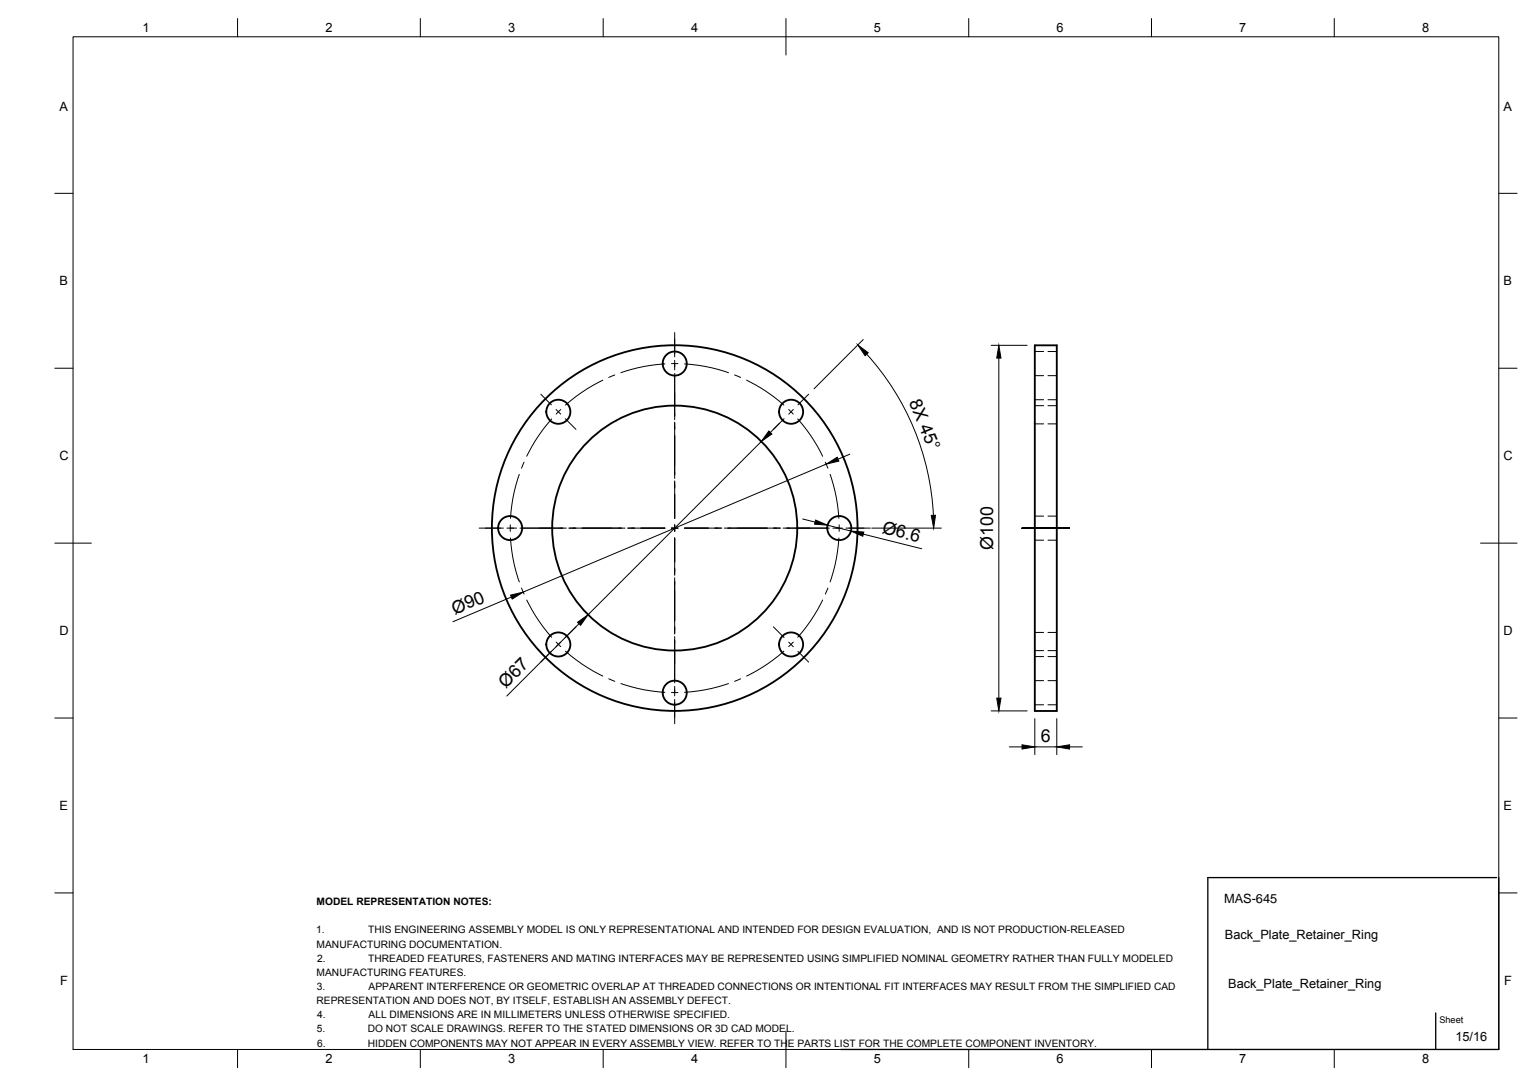
ISO-10303-21;
HEADER;
FILE_DESCRIPTION((''),'2;1');
FILE_NAME('Back_Plate_Retainer_Ring.step','2026-10-09T10:54:55-07:00',(''),(''),'','','');
FILE_SCHEMA (('AUTOMOTIVE_DESIGN { 1 0 10303 214 3 1 1 }'));
ENDSEC;
DATA;
#10=MECHANICAL_DESIGN_GEOMETRIC_PRESENTATION_REPRESENTATION('',(#608),#63824);
#578=SHAPE_REPRESENTATION_RELATIONSHIP('SRR','None',#63892,#593) ;
#593=ADVANCED_BREP_SHAPE_REPRESENTATION('',(#623),#63822) ;
#608=STYLED_ITEM('',(#63963),#623) ;
#623=MANIFOLD_SOLID_BREP('Body1',#15507) ;
#796=FACE_BOUND('',#3425,.T.) ;
#797=FACE_BOUND('',#3426,.T.) ;
#798=FACE_BOUND('',#3427,.T.) ;
#799=FACE_BOUND('',#3428,.T.) ;
#800=FACE_BOUND('',#3429,.T.) ;
#801=FACE_BOUND('',#3430,.T.) ;
#802=FACE_BOUND('',#3431,.T.) ;
#803=FACE_BOUND('',#3432,.T.) ;
#804=FACE_BOUND('',#3433,.T.) ;
#805=FACE_BOUND('',#3435,.T.) ;
#806=FACE_BOUND('',#3436,.T.) ;
#807=FACE_BOUND('',#3437,.T.) ;
#808=FACE_BOUND('',#3438,.T.) ;
#809=FACE_BOUND('',#3439,.T.) ;
#810=FACE_BOUND('',#3440,.T.) ;
#811=FACE_BOUND('',#3441,.T.) ;
#812=FACE_BOUND('',#3442,.T.) ;
#813=FACE_BOUND('',#3443,.T.) ;
#1112=PLANE('',#17850) ;
#1113=PLANE('',#17851) ;
#1525=CYLINDRICAL_SURFACE('',#17820,3.3) ;
#1526=CYLINDRICAL_SURFACE('',#17823,3.3) ;
#1527=CYLINDRICAL_SURFACE('',#17826,3.3) ;
#1528=CYLINDRICAL_SURFACE('',#17829,3.3) ;
#1529=CYLINDRICAL_SURFACE('',#17832,3.3) ;
#1530=CYLINDRICAL_SURFACE('',#17835,3.3) ;
#1531=CYLINDRICAL_SURFACE('',#17838,3.3) ;
#1532=CYLINDRICAL_SURFACE('',#17841,3.3) ;
#1533=CYLINDRICAL_SURFACE('',#17844,33.5) ;
#1534=CYLINDRICAL_SURFACE('',#17847,50.) ;
#2382=FACE_OUTER_BOUND('',#3414,.T.) ;
#2383=FACE_OUTER_BOUND('',#3415,.T.) ;
#2384=FACE_OUTER_BOUND('',#3416,.T.) ;
#2385=FACE_OUTER_BOUND('',#3417,.T.) ;
#2386=FACE_OUTER_BOUND('',#3418,.T.) ;
#2387=FACE_OUTER_BOUND('',#3419,.T.) ;
#2388=FACE_OUTER_BOUND('',#3420,.T.) ;
#2389=FACE_OUTER_BOUND('',#3421,.T.) ;
#2390=FACE_OUTER_BOUND('',#3422,.T.) ;
#2391=FACE_OUTER_BOUND('',#3423,.T.) ;
#2392=FACE_OUTER_BOUND('',#3424,.T.) ;
#2393=FACE_OUTER_BOUND('',#3434,.T.) ;
#3414=EDGE_LOOP('',(#14376,#14377,#14378,#14379)) ;
#3415=EDGE_LOOP('',(#14380,#14381,#14382,#14383)) ;
#3416=EDGE_LOOP('',(#14384,#14385,#14386,#14387)) ;
#3417=EDGE_LOOP('',(#14388,#14389,#14390,#14391)) ;
#3418=EDGE_LOOP('',(#14392,#14393,#14394,#14395)) ;
#3419=EDGE_LOOP('',(#14396,#14397,#14398,#14399)) ;
#3420=EDGE_LOOP('',(#14400,#14401,#14402,#14403)) ;
#3421=EDGE_LOOP('',(#14404,#14405,#14406,#14407)) ;
#3422=EDGE_LOOP('',(#14408,#14409,#14410,#14411)) ;
#3423=EDGE_LOOP('',(#14412,#14413,#14414,#14415)) ;
#3424=EDGE_LOOP('',(#14416)) ;
#3425=EDGE_LOOP('',(#14417)) ;
#3426=EDGE_LOOP('',(#14418)) ;
#3427=EDGE_LOOP('',(#14419)) ;
#3428=EDGE_LOOP('',(#14420)) ;
#3429=EDGE_LOOP('',(#14421)) ;
#3430=EDGE_LOOP('',(#14422)) ;
#3431=EDGE_LOOP('',(#14423)) ;
#3432=EDGE_LOOP('',(#14424)) ;
#3433=EDGE_LOOP('',(#14425)) ;
#3434=EDGE_LOOP('',(#14426)) ;
#3435=EDGE_LOOP('',(#14427)) ;
#3436=EDGE_LOOP('',(#14428)) ;
#3437=EDGE_LOOP('',(#14429)) ;
#3438=EDGE_LOOP('',(#14430)) ;
#3439=EDGE_LOOP('',(#14431)) ;
#3440=EDGE_LOOP('',(#14432)) ;
#3441=EDGE_LOOP('',(#14433)) ;
#3442=EDGE_LOOP('',(#14434)) ;
#3443=EDGE_LOOP('',(#14435)) ;
#4650=CIRCLE('',#17821,3.3) ;
#4651=CIRCLE('',#17822,3.3) ;
#4652=CIRCLE('',#17824,3.3) ;
#4653=CIRCLE('',#17825,3.3) ;
#4654=CIRCLE('',#17827,3.3) ;
#4655=CIRCLE('',#17828,3.3) ;
#4656=CIRCLE('',#17830,3.3) ;
#4657=CIRCLE('',#17831,3.3) ;
#4658=CIRCLE('',#17833,3.3) ;
#4659=CIRCLE('',#17834,3.3) ;
#4660=CIRCLE('',#17836,3.3) ;
#4661=CIRCLE('',#17837,3.3) ;
#4662=CIRCLE('',#17839,3.3) ;
#4663=CIRCLE('',#17840,3.3) ;
#4664=CIRCLE('',#17842,3.3) ;
#4665=CIRCLE('',#17843,3.3) ;
#4666=CIRCLE('',#17845,33.5) ;
#4667=CIRCLE('',#17846,33.5) ;
#4668=CIRCLE('',#17848,50.) ;
#4669=CIRCLE('',#17849,50.) ;
#5326=LINE('',#63653,#5982) ;
#5327=LINE('',#63659,#5983) ;
#5328=LINE('',#63665,#5984) ;
#5329=LINE('',#63671,#5985) ;
#5330=LINE('',#63677,#5986) ;
#5331=LINE('',#63683,#5987) ;
#5332=LINE('',#63689,#5988) ;
#5333=LINE('',#63695,#5989) ;
#5334=LINE('',#63701,#5990) ;
#5335=LINE('',#63707,#5991) ;
#5982=VECTOR('',#22832,3.3) ;
#5983=VECTOR('',#22839,3.3) ;
#5984=VECTOR('',#22846,3.3) ;
#5985=VECTOR('',#22853,3.3) ;
#5986=VECTOR('',#22860,3.3) ;
#5987=VECTOR('',#22867,3.3) ;
#5988=VECTOR('',#22874,3.3) ;
#5989=VECTOR('',#22881,3.3) ;
#5990=VECTOR('',#22888,33.5) ;
#5991=VECTOR('',#22895,50.) ;
#7415=VERTEX_POINT('',#63650) ;
#7416=VERTEX_POINT('',#63652) ;
#7417=VERTEX_POINT('',#63656) ;
#7418=VERTEX_POINT('',#63658) ;
#7419=VERTEX_POINT('',#63662) ;
#7420=VERTEX_POINT('',#63664) ;
#7421=VERTEX_POINT('',#63668) ;
#7422=VERTEX_POINT('',#63670) ;
#7423=VERTEX_POINT('',#63674) ;
#7424=VERTEX_POINT('',#63676) ;
#7425=VERTEX_POINT('',#63680) ;
#7426=VERTEX_POINT('',#63682) ;
#7427=VERTEX_POINT('',#63686) ;
#7428=VERTEX_POINT('',#63688) ;
#7429=VERTEX_POINT('',#63692) ;
#7430=VERTEX_POINT('',#63694) ;
#7431=VERTEX_POINT('',#63698) ;
#7432=VERTEX_POINT('',#63700) ;
#7433=VERTEX_POINT('',#63704) ;
#7434=VERTEX_POINT('',#63706) ;
#9742=EDGE_CURVE('',#7415,#7415,#4650,.T.) ;
#9743=EDGE_CURVE('',#7415,#7416,#5326,.T.) ;
#9744=EDGE_CURVE('',#7416,#7416,#4651,.T.) ;
#9745=EDGE_CURVE('',#7417,#7417,#4652,.T.) ;
#9746=EDGE_CURVE('',#7417,#7418,#5327,.T.) ;
#9747=EDGE_CURVE('',#7418,#7418,#4653,.T.) ;
#9748=EDGE_CURVE('',#7419,#7419,#4654,.T.) ;
#9749=EDGE_CURVE('',#7419,#7420,#5328,.T.) ;
#9750=EDGE_CURVE('',#7420,#7420,#4655,.T.) ;
#9751=EDGE_CURVE('',#7421,#7421,#4656,.T.) ;
#9752=EDGE_CURVE('',#7421,#7422,#5329,.T.) ;
#9753=EDGE_CURVE('',#7422,#7422,#4657,.T.) ;
#9754=EDGE_CURVE('',#7423,#7423,#4658,.T.) ;
#9755=EDGE_CURVE('',#7423,#7424,#5330,.T.) ;
#9756=EDGE_CURVE('',#7424,#7424,#4659,.T.) ;
#9757=EDGE_CURVE('',#7425,#7425,#4660,.T.) ;
#9758=EDGE_CURVE('',#7425,#7426,#5331,.T.) ;
#9759=EDGE_CURVE('',#7426,#7426,#4661,.T.) ;
#9760=EDGE_CURVE('',#7427,#7427,#4662,.T.) ;
#9761=EDGE_CURVE('',#7427,#7428,#5332,.T.) ;
#9762=EDGE_CURVE('',#7428,#7428,#4663,.T.) ;
#9763=EDGE_CURVE('',#7429,#7429,#4664,.T.) ;
#9764=EDGE_CURVE('',#7429,#7430,#5333,.T.) ;
#9765=EDGE_CURVE('',#7430,#7430,#4665,.T.) ;
#9766=EDGE_CURVE('',#7431,#7431,#4666,.T.) ;
#9767=EDGE_CURVE('',#7431,#7432,#5334,.T.) ;
#9768=EDGE_CURVE('',#7432,#7432,#4667,.T.) ;
#9769=EDGE_CURVE('',#7433,#7433,#4668,.T.) ;
#9770=EDGE_CURVE('',#7433,#7434,#5335,.T.) ;
#9771=EDGE_CURVE('',#7434,#7434,#4669,.T.) ;
#14376=ORIENTED_EDGE('',*,*,#9742,.F.) ;
#14377=ORIENTED_EDGE('',*,*,#9743,.T.) ;
#14378=ORIENTED_EDGE('',*,*,#9744,.F.) ;
#14379=ORIENTED_EDGE('',*,*,#9743,.F.) ;
#14380=ORIENTED_EDGE('',*,*,#9745,.F.) ;
#14381=ORIENTED_EDGE('',*,*,#9746,.T.) ;
#14382=ORIENTED_EDGE('',*,*,#9747,.F.) ;
#14383=ORIENTED_EDGE('',*,*,#9746,.F.) ;
#14384=ORIENTED_EDGE('',*,*,#9748,.F.) ;
#14385=ORIENTED_EDGE('',*,*,#9749,.T.) ;
#14386=ORIENTED_EDGE('',*,*,#9750,.F.) ;
#14387=ORIENTED_EDGE('',*,*,#9749,.F.) ;
#14388=ORIENTED_EDGE('',*,*,#9751,.F.) ;
#14389=ORIENTED_EDGE('',*,*,#9752,.T.) ;
#14390=ORIENTED_EDGE('',*,*,#9753,.F.) ;
#14391=ORIENTED_EDGE('',*,*,#9752,.F.) ;
#14392=ORIENTED_EDGE('',*,*,#9754,.F.) ;
#14393=ORIENTED_EDGE('',*,*,#9755,.T.) ;
#14394=ORIENTED_EDGE('',*,*,#9756,.F.) ;
#14395=ORIENTED_EDGE('',*,*,#9755,.F.) ;
#14396=ORIENTED_EDGE('',*,*,#9757,.F.) ;
#14397=ORIENTED_EDGE('',*,*,#9758,.T.) ;
#14398=ORIENTED_EDGE('',*,*,#9759,.F.) ;
#14399=ORIENTED_EDGE('',*,*,#9758,.F.) ;
#14400=ORIENTED_EDGE('',*,*,#9760,.F.) ;
#14401=ORIENTED_EDGE('',*,*,#9761,.T.) ;
#14402=ORIENTED_EDGE('',*,*,#9762,.F.) ;
#14403=ORIENTED_EDGE('',*,*,#9761,.F.) ;
#14404=ORIENTED_EDGE('',*,*,#9763,.F.) ;
#14405=ORIENTED_EDGE('',*,*,#9764,.T.) ;
#14406=ORIENTED_EDGE('',*,*,#9765,.F.) ;
#14407=ORIENTED_EDGE('',*,*,#9764,.F.) ;
#14408=ORIENTED_EDGE('',*,*,#9766,.F.) ;
#14409=ORIENTED_EDGE('',*,*,#9767,.T.) ;
#14410=ORIENTED_EDGE('',*,*,#9768,.F.) ;
#14411=ORIENTED_EDGE('',*,*,#9767,.F.) ;
#14412=ORIENTED_EDGE('',*,*,#9769,.F.) ;
#14413=ORIENTED_EDGE('',*,*,#9770,.T.) ;
#14414=ORIENTED_EDGE('',*,*,#9771,.F.) ;
#14415=ORIENTED_EDGE('',*,*,#9770,.F.) ;
#14416=ORIENTED_EDGE('',*,*,#9771,.T.) ;
#14417=ORIENTED_EDGE('',*,*,#9744,.T.) ;
#14418=ORIENTED_EDGE('',*,*,#9747,.T.) ;
#14419=ORIENTED_EDGE('',*,*,#9750,.T.) ;
#14420=ORIENTED_EDGE('',*,*,#9753,.T.) ;
#14421=ORIENTED_EDGE('',*,*,#9756,.T.) ;
#14422=ORIENTED_EDGE('',*,*,#9759,.T.) ;
#14423=ORIENTED_EDGE('',*,*,#9762,.T.) ;
#14424=ORIENTED_EDGE('',*,*,#9765,.T.) ;
#14425=ORIENTED_EDGE('',*,*,#9766,.T.) ;
#14426=ORIENTED_EDGE('',*,*,#9769,.T.) ;
#14427=ORIENTED_EDGE('',*,*,#9742,.T.) ;
#14428=ORIENTED_EDGE('',*,*,#9745,.T.) ;
#14429=ORIENTED_EDGE('',*,*,#9748,.T.) ;
#14430=ORIENTED_EDGE('',*,*,#9751,.T.) ;
#14431=ORIENTED_EDGE('',*,*,#9754,.T.) ;
#14432=ORIENTED_EDGE('',*,*,#9757,.T.) ;
#14433=ORIENTED_EDGE('',*,*,#9760,.T.) ;
#14434=ORIENTED_EDGE('',*,*,#9763,.T.) ;
#14435=ORIENTED_EDGE('',*,*,#9768,.T.) ;
#15470=ADVANCED_FACE('',(#2382),#1525,.F.) ;
#15471=ADVANCED_FACE('',(#2383),#1526,.F.) ;
#15472=ADVANCED_FACE('',(#2384),#1527,.F.) ;
#15473=ADVANCED_FACE('',(#2385),#1528,.F.) ;
#15474=ADVANCED_FACE('',(#2386),#1529,.F.) ;
#15475=ADVANCED_FACE('',(#2387),#1530,.F.) ;
#15476=ADVANCED_FACE('',(#2388),#1531,.F.) ;
#15477=ADVANCED_FACE('',(#2389),#1532,.F.) ;
#15478=ADVANCED_FACE('',(#2390),#1533,.F.) ;
#15479=ADVANCED_FACE('',(#2391),#1534,.T.) ;
#15480=ADVANCED_FACE('',(#2392,#796,#797,#798,#799,#800,#801,#802,#803,
#804),#1112,.F.) ;
#15481=ADVANCED_FACE('',(#2393,#805,#806,#807,#808,#809,#810,#811,#812,
#813),#1113,.T.) ;
#15507=CLOSED_SHELL('',(#15470,#15471,#15472,#15473,#15474,#15475,#15476,
#15477,#15478,#15479,#15480,#15481)) ;
#17819=AXIS2_PLACEMENT_3D('',#63648,#22826,#22827) ;
#17820=AXIS2_PLACEMENT_3D('',#63649,#22828,#22829) ;
#17821=AXIS2_PLACEMENT_3D('',#63651,#22830,#22831) ;
#17822=AXIS2_PLACEMENT_3D('',#63654,#22833,#22834) ;
#17823=AXIS2_PLACEMENT_3D('',#63655,#22835,#22836) ;
#17824=AXIS2_PLACEMENT_3D('',#63657,#22837,#22838) ;
#17825=AXIS2_PLACEMENT_3D('',#63660,#22840,#22841) ;
#17826=AXIS2_PLACEMENT_3D('',#63661,#22842,#22843) ;
#17827=AXIS2_PLACEMENT_3D('',#63663,#22844,#22845) ;
#17828=AXIS2_PLACEMENT_3D('',#63666,#22847,#22848) ;
#17829=AXIS2_PLACEMENT_3D('',#63667,#22849,#22850) ;
#17830=AXIS2_PLACEMENT_3D('',#63669,#22851,#22852) ;
#17831=AXIS2_PLACEMENT_3D('',#63672,#22854,#22855) ;
#17832=AXIS2_PLACEMENT_3D('',#63673,#22856,#22857) ;
#17833=AXIS2_PLACEMENT_3D('',#63675,#22858,#22859) ;
#17834=AXIS2_PLACEMENT_3D('',#63678,#22861,#22862) ;
#17835=AXIS2_PLACEMENT_3D('',#63679,#22863,#22864) ;
#17836=AXIS2_PLACEMENT_3D('',#63681,#22865,#22866) ;
#17837=AXIS2_PLACEMENT_3D('',#63684,#22868,#22869) ;
#17838=AXIS2_PLACEMENT_3D('',#63685,#22870,#22871) ;
#17839=AXIS2_PLACEMENT_3D('',#63687,#22872,#22873) ;
#17840=AXIS2_PLACEMENT_3D('',#63690,#22875,#22876) ;
#17841=AXIS2_PLACEMENT_3D('',#63691,#22877,#22878) ;
#17842=AXIS2_PLACEMENT_3D('',#63693,#22879,#22880) ;
#17843=AXIS2_PLACEMENT_3D('',#63696,#22882,#22883) ;
#17844=AXIS2_PLACEMENT_3D('',#63697,#22884,#22885) ;
#17845=AXIS2_PLACEMENT_3D('',#63699,#22886,#22887) ;
#17846=AXIS2_PLACEMENT_3D('',#63702,#22889,#22890) ;
#17847=AXIS2_PLACEMENT_3D('',#63703,#22891,#22892) ;
#17848=AXIS2_PLACEMENT_3D('',#63705,#22893,#22894) ;
#17849=AXIS2_PLACEMENT_3D('',#63708,#22896,#22897) ;
#17850=AXIS2_PLACEMENT_3D('',#63709,#22898,#22899) ;
#17851=AXIS2_PLACEMENT_3D('',#63710,#22900,#22901) ;
#22826=DIRECTION('axis',(0.,0.,1.)) ;
#22827=DIRECTION('refdir',(1.,0.,0.)) ;
#22828=DIRECTION('center_axis',(0.,0.,1.)) ;
#22829=DIRECTION('ref_axis',(-1.,0.,0.)) ;
#22830=DIRECTION('center_axis',(0.,0.,1.)) ;
#22831=DIRECTION('ref_axis',(-1.,0.,0.)) ;
#22832=DIRECTION('',(0.,0.,1.)) ;
#22833=DIRECTION('center_axis',(0.,0.,-1.)) ;
#22834=DIRECTION('ref_axis',(-1.,0.,0.)) ;
#22835=DIRECTION('center_axis',(0.,0.,1.)) ;
#22836=DIRECTION('ref_axis',(-1.,0.,0.)) ;
#22837=DIRECTION('center_axis',(0.,0.,1.)) ;
#22838=DIRECTION('ref_axis',(-1.,0.,0.)) ;
#22839=DIRECTION('',(0.,0.,1.)) ;
#22840=DIRECTION('center_axis',(0.,0.,-1.)) ;
#22841=DIRECTION('ref_axis',(-1.,0.,0.)) ;
#22842=DIRECTION('center_axis',(0.,0.,1.)) ;
#22843=DIRECTION('ref_axis',(-1.,0.,0.)) ;
#22844=DIRECTION('center_axis',(0.,0.,1.)) ;
#22845=DIRECTION('ref_axis',(-1.,0.,0.)) ;
#22846=DIRECTION('',(0.,0.,1.)) ;
#22847=DIRECTION('center_axis',(0.,0.,-1.)) ;
#22848=DIRECTION('ref_axis',(-1.,0.,0.)) ;
#22849=DIRECTION('center_axis',(0.,0.,1.)) ;
#22850=DIRECTION('ref_axis',(-1.,0.,0.)) ;
#22851=DIRECTION('center_axis',(0.,0.,1.)) ;
#22852=DIRECTION('ref_axis',(-1.,0.,0.)) ;
#22853=DIRECTION('',(0.,0.,1.)) ;
#22854=DIRECTION('center_axis',(0.,0.,-1.)) ;
#22855=DIRECTION('ref_axis',(-1.,0.,0.)) ;
#22856=DIRECTION('center_axis',(0.,0.,1.)) ;
#22857=DIRECTION('ref_axis',(-1.,0.,0.)) ;
#22858=DIRECTION('center_axis',(0.,0.,1.)) ;
#22859=DIRECTION('ref_axis',(-1.,0.,0.)) ;
#22860=DIRECTION('',(0.,0.,1.)) ;
#22861=DIRECTION('center_axis',(0.,0.,-1.)) ;
#22862=DIRECTION('ref_axis',(-1.,0.,0.)) ;
#22863=DIRECTION('center_axis',(0.,0.,1.)) ;
#22864=DIRECTION('ref_axis',(-1.,0.,0.)) ;
#22865=DIRECTION('center_axis',(0.,0.,1.)) ;
#22866=DIRECTION('ref_axis',(-1.,0.,0.)) ;
#22867=DIRECTION('',(0.,0.,1.)) ;
#22868=DIRECTION('center_axis',(0.,0.,-1.)) ;
#22869=DIRECTION('ref_axis',(-1.,0.,0.)) ;
#22870=DIRECTION('center_axis',(0.,0.,1.)) ;
#22871=DIRECTION('ref_axis',(-1.,0.,0.)) ;
#22872=DIRECTION('center_axis',(0.,0.,1.)) ;
#22873=DIRECTION('ref_axis',(-1.,0.,0.)) ;
#22874=DIRECTION('',(0.,0.,1.)) ;
#22875=DIRECTION('center_axis',(0.,0.,-1.)) ;
#22876=DIRECTION('ref_axis',(-1.,0.,0.)) ;
#22877=DIRECTION('center_axis',(0.,0.,1.)) ;
#22878=DIRECTION('ref_axis',(-1.,0.,0.)) ;
#22879=DIRECTION('center_axis',(0.,0.,1.)) ;
#22880=DIRECTION('ref_axis',(-1.,0.,0.)) ;
#22881=DIRECTION('',(0.,0.,1.)) ;
#22882=DIRECTION('center_axis',(0.,0.,-1.)) ;
#22883=DIRECTION('ref_axis',(-1.,0.,0.)) ;
#22884=DIRECTION('center_axis',(0.,0.,-1.)) ;
#22885=DIRECTION('ref_axis',(1.,0.,0.)) ;
#22886=DIRECTION('center_axis',(0.,0.,-1.)) ;
#22887=DIRECTION('ref_axis',(1.,0.,0.)) ;
#22888=DIRECTION('',(0.,0.,-1.)) ;
#22889=DIRECTION('center_axis',(0.,0.,1.)) ;
#22890=DIRECTION('ref_axis',(1.,0.,0.)) ;
#22891=DIRECTION('center_axis',(0.,0.,-1.)) ;
#22892=DIRECTION('ref_axis',(1.,0.,0.)) ;
#22893=DIRECTION('center_axis',(0.,0.,-1.)) ;
#22894=DIRECTION('ref_axis',(1.,0.,0.)) ;
#22895=DIRECTION('',(0.,0.,1.)) ;
#22896=DIRECTION('center_axis',(0.,0.,1.)) ;
#22897=DIRECTION('ref_axis',(1.,0.,0.)) ;
#22898=DIRECTION('center_axis',(0.,0.,-1.)) ;
#22899=DIRECTION('ref_axis',(-1.,0.,0.)) ;
#22900=DIRECTION('center_axis',(0.,0.,-1.)) ;
#22901=DIRECTION('ref_axis',(-1.,0.,0.)) ;
#63648=CARTESIAN_POINT('',(0.,0.,0.)) ;
#63649=CARTESIAN_POINT('Origin',(45.,354.45,-22.)) ;
#63650=CARTESIAN_POINT('',(48.3,354.45,-30.)) ;
#63651=CARTESIAN_POINT('Origin',(45.,354.45,-30.)) ;
#63652=CARTESIAN_POINT('',(48.3,354.45,-24.)) ;
#63653=CARTESIAN_POINT('',(48.3,354.45,-22.)) ;
#63654=CARTESIAN_POINT('Origin',(45.,354.45,-24.)) ;
#63655=CARTESIAN_POINT('Origin',(-5.51091059616309E-15,399.45,-22.)) ;
#63656=CARTESIAN_POINT('',(3.29999999999999,399.45,-30.)) ;
#63657=CARTESIAN_POINT('Origin',(-5.51091059616309E-15,399.45,-30.)) ;
#63658=CARTESIAN_POINT('',(3.29999999999999,399.45,-24.)) ;
#63659=CARTESIAN_POINT('',(3.29999999999999,399.45,-22.)) ;
#63660=CARTESIAN_POINT('Origin',(-5.51091059616309E-15,399.45,-24.)) ;
#63661=CARTESIAN_POINT('Origin',(-45.,354.45,-22.)) ;
#63662=CARTESIAN_POINT('',(-41.7,354.45,-30.)) ;
#63663=CARTESIAN_POINT('Origin',(-45.,354.45,-30.)) ;
#63664=CARTESIAN_POINT('',(-41.7,354.45,-24.)) ;
#63665=CARTESIAN_POINT('',(-41.7,354.45,-22.)) ;
#63666=CARTESIAN_POINT('Origin',(-45.,354.45,-24.)) ;
#63667=CARTESIAN_POINT('Origin',(0.,309.45,-22.)) ;
#63668=CARTESIAN_POINT('',(3.3,309.45,-30.)) ;
#63669=CARTESIAN_POINT('Origin',(0.,309.45,-30.)) ;
#63670=CARTESIAN_POINT('',(3.3,309.45,-24.)) ;
#63671=CARTESIAN_POINT('',(3.3,309.45,-22.)) ;
#63672=CARTESIAN_POINT('Origin',(0.,309.45,-24.)) ;
#63673=CARTESIAN_POINT('Origin',(-31.8198051533946,322.630194846605,-22.)) ;
#63674=CARTESIAN_POINT('',(-28.5198051533946,322.630194846605,-30.)) ;
#63675=CARTESIAN_POINT('Origin',(-31.8198051533946,322.630194846605,-30.)) ;
#63676=CARTESIAN_POINT('',(-28.5198051533946,322.630194846605,-24.)) ;
#63677=CARTESIAN_POINT('',(-28.5198051533946,322.630194846605,-22.)) ;
#63678=CARTESIAN_POINT('Origin',(-31.8198051533946,322.630194846605,-24.)) ;
#63679=CARTESIAN_POINT('Origin',(-31.8198051533946,386.269805153395,-22.)) ;
#63680=CARTESIAN_POINT('',(-28.5198051533946,386.269805153395,-30.)) ;
#63681=CARTESIAN_POINT('Origin',(-31.8198051533946,386.269805153395,-30.)) ;
#63682=CARTESIAN_POINT('',(-28.5198051533946,386.269805153395,-24.)) ;
#63683=CARTESIAN_POINT('',(-28.5198051533946,386.269805153395,-22.)) ;
#63684=CARTESIAN_POINT('Origin',(-31.8198051533946,386.269805153395,-24.)) ;
#63685=CARTESIAN_POINT('Origin',(31.8198051533946,386.269805153395,-22.)) ;
#63686=CARTESIAN_POINT('',(35.1198051533946,386.269805153395,-30.)) ;
#63687=CARTESIAN_POINT('Origin',(31.8198051533946,386.269805153395,-30.)) ;
#63688=CARTESIAN_POINT('',(35.1198051533946,386.269805153395,-24.)) ;
#63689=CARTESIAN_POINT('',(35.1198051533946,386.269805153395,-22.)) ;
#63690=CARTESIAN_POINT('Origin',(31.8198051533946,386.269805153395,-24.)) ;
#63691=CARTESIAN_POINT('Origin',(31.8198051533946,322.630194846605,-22.)) ;
#63692=CARTESIAN_POINT('',(35.1198051533946,322.630194846605,-30.)) ;
#63693=CARTESIAN_POINT('Origin',(31.8198051533946,322.630194846605,-30.)) ;
#63694=CARTESIAN_POINT('',(35.1198051533946,322.630194846605,-24.)) ;
#63695=CARTESIAN_POINT('',(35.1198051533946,322.630194846605,-22.)) ;
#63696=CARTESIAN_POINT('Origin',(31.8198051533946,322.630194846605,-24.)) ;
#63697=CARTESIAN_POINT('Origin',(0.,354.45,-24.)) ;
#63698=CARTESIAN_POINT('',(-33.5,354.45,-24.)) ;
#63699=CARTESIAN_POINT('Origin',(0.,354.45,-24.)) ;
#63700=CARTESIAN_POINT('',(-33.5,354.45,-30.)) ;
#63701=CARTESIAN_POINT('',(-33.5,354.45,-24.)) ;
#63702=CARTESIAN_POINT('Origin',(0.,354.45,-30.)) ;
#63703=CARTESIAN_POINT('Origin',(0.,354.45,-24.)) ;
#63704=CARTESIAN_POINT('',(-50.,354.45,-30.)) ;
#63705=CARTESIAN_POINT('Origin',(0.,354.45,-30.)) ;
#63706=CARTESIAN_POINT('',(-50.,354.45,-24.)) ;
#63707=CARTESIAN_POINT('',(-50.,354.45,-24.)) ;
#63708=CARTESIAN_POINT('Origin',(0.,354.45,-24.)) ;
#63709=CARTESIAN_POINT('Origin',(0.,354.45,-24.)) ;
#63710=CARTESIAN_POINT('Origin',(0.,354.45,-30.)) ;
#63805=UNCERTAINTY_MEASURE_WITH_UNIT(LENGTH_MEASURE(0.01),#63825,
'DISTANCE_ACCURACY_VALUE',
'Maximum model space distance between geometric entities at asserted c
onnectivities') ;
#63807=UNCERTAINTY_MEASURE_WITH_UNIT(LENGTH_MEASURE(0.01),#63825,
'DISTANCE_ACCURACY_VALUE',
'Maximum model space distance between geometric entities at asserted c
onnectivities') ;
#63822=(
GEOMETRIC_REPRESENTATION_CONTEXT(3)
GLOBAL_UNCERTAINTY_ASSIGNED_CONTEXT((#63805))
GLOBAL_UNIT_ASSIGNED_CONTEXT((#63825,#63827,#63828))
REPRESENTATION_CONTEXT('','3D')
) ;
#63824=(
GEOMETRIC_REPRESENTATION_CONTEXT(3)
GLOBAL_UNCERTAINTY_ASSIGNED_CONTEXT((#63807))
GLOBAL_UNIT_ASSIGNED_CONTEXT((#63825,#63827,#63828))
REPRESENTATION_CONTEXT('','3D')
) ;
#63825=(
LENGTH_UNIT()
NAMED_UNIT(*)
SI_UNIT(.MILLI.,.METRE.)
) ;
#63827=(
NAMED_UNIT(*)
PLANE_ANGLE_UNIT()
SI_UNIT($,.RADIAN.)
) ;
#63828=(
NAMED_UNIT(*)
SI_UNIT($,.STERADIAN.)
SOLID_ANGLE_UNIT()
) ;
#63843=SHAPE_DEFINITION_REPRESENTATION(#63859,#63892) ;
#63859=PRODUCT_DEFINITION_SHAPE('',$,#63909) ;
#63892=SHAPE_REPRESENTATION('',(#17819),#63822) ;
#63894=PRODUCT_DEFINITION_CONTEXT('part definition',#63944,'design') ;
#63909=PRODUCT_DEFINITION('Back_Plate_Retainer_Ring',
'Back_Plate_Retainer_Ring',#63925,#63894) ;
#63925=PRODUCT_DEFINITION_FORMATION('',$,#63960) ;
#63944=APPLICATION_CONTEXT(
'Core Data for Automotive Mechanical Design Process') ;
#63945=PRODUCT_CONTEXT('part definition',#63944,'mechanical') ;
#63960=PRODUCT('Back_Plate_Retainer_Ring','Back_Plate_Retainer_Ring',$,
(#63945)) ;
#63963=PRESENTATION_STYLE_ASSIGNMENT((#63968)) ;
#63968=SURFACE_STYLE_USAGE(.BOTH.,#63973) ;
#63973=SURFACE_SIDE_STYLE('',(#63978)) ;
#63978=SURFACE_STYLE_FILL_AREA(#63983) ;
#63983=FILL_AREA_STYLE('Opaque(160,160,160)',(#63988)) ;
#63988=FILL_AREA_STYLE_COLOUR('Opaque(160,160,160)',#63993) ;
#63993=COLOUR_RGB('Opaque(160,160,160)', 0.09019608, 0.27058824, 0.51372549) ;
ENDSEC;
END-ISO-10303-21;
